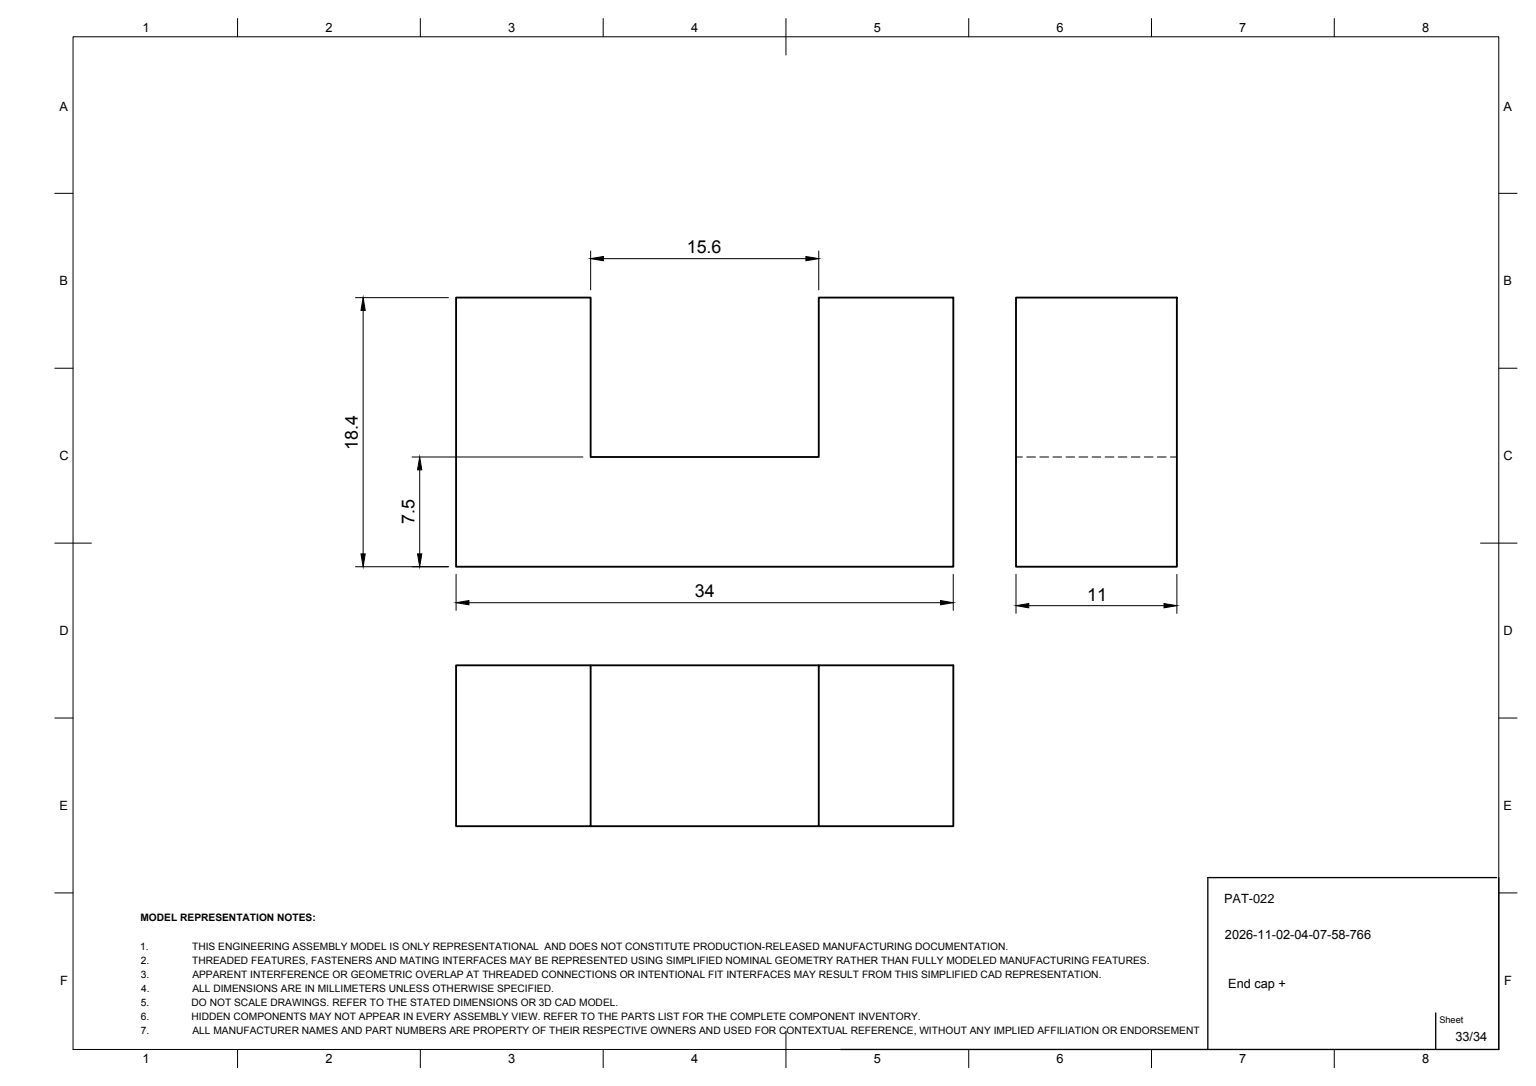
ISO-10303-21;
HEADER;
/* Generated by software containing ST-Developer
 * from STEP Tools, Inc. (www.steptools.com) 
 */

FILE_DESCRIPTION(
/* description */ ('Chute with adjustable gate'),
/* implementation_level */ '2;1');

FILE_NAME(
/* name */ 'End cap +.step',
/* time_stamp */ '2026-10-27T10:52:28-07:00',
/* author */ (''),
/* organization */ (''),
/* preprocessor_version */ 'ST-DEVELOPER v20.2',
/* originating_system */ 'Autodesk Translation Framework v15.17.0.0',
/* authorisation */ '');

FILE_SCHEMA (('AUTOMOTIVE_DESIGN { 1 0 10303 214 3 1 1 }'));
ENDSEC;

DATA;
#10=MECHANICAL_DESIGN_GEOMETRIC_PRESENTATION_REPRESENTATION('',(#442),#13094);
#378=SHAPE_REPRESENTATION_RELATIONSHIP('SRR','None',#13281,#410);
#410=ADVANCED_BREP_SHAPE_REPRESENTATION('',(#472),#13090);
#442=STYLED_ITEM('',(#13488),#472);
#472=MANIFOLD_SOLID_BREP('Body1',#7627);
#872=PLANE('',#8549);
#873=PLANE('',#8550);
#874=PLANE('',#8551);
#875=PLANE('',#8552);
#876=PLANE('',#8553);
#877=PLANE('',#8554);
#878=PLANE('',#8555);
#879=PLANE('',#8556);
#880=PLANE('',#8557);
#881=PLANE('',#8558);
#1276=FACE_OUTER_BOUND('',#1805,.T.);
#1277=FACE_OUTER_BOUND('',#1806,.T.);
#1278=FACE_OUTER_BOUND('',#1807,.T.);
#1279=FACE_OUTER_BOUND('',#1808,.T.);
#1280=FACE_OUTER_BOUND('',#1809,.T.);
#1281=FACE_OUTER_BOUND('',#1810,.T.);
#1282=FACE_OUTER_BOUND('',#1811,.T.);
#1283=FACE_OUTER_BOUND('',#1812,.T.);
#1284=FACE_OUTER_BOUND('',#1813,.T.);
#1285=FACE_OUTER_BOUND('',#1814,.T.);
#1805=EDGE_LOOP('',(#6886,#6887,#6888,#6889));
#1806=EDGE_LOOP('',(#6890,#6891,#6892,#6893));
#1807=EDGE_LOOP('',(#6894,#6895,#6896,#6897));
#1808=EDGE_LOOP('',(#6898,#6899,#6900,#6901));
#1809=EDGE_LOOP('',(#6902,#6903,#6904,#6905));
#1810=EDGE_LOOP('',(#6906,#6907,#6908,#6909));
#1811=EDGE_LOOP('',(#6910,#6911,#6912,#6913));
#1812=EDGE_LOOP('',(#6914,#6915,#6916,#6917));
#1813=EDGE_LOOP('',(#6918,#6919,#6920,#6921,#6922,#6923,#6924,#6925));
#1814=EDGE_LOOP('',(#6926,#6927,#6928,#6929,#6930,#6931,#6932,#6933));
#2542=LINE('',#12709,#3319);
#2543=LINE('',#12711,#3320);
#2544=LINE('',#12713,#3321);
#2545=LINE('',#12714,#3322);
#2546=LINE('',#12717,#3323);
#2547=LINE('',#12719,#3324);
#2548=LINE('',#12720,#3325);
#2549=LINE('',#12723,#3326);
#2550=LINE('',#12725,#3327);
#2551=LINE('',#12726,#3328);
#2552=LINE('',#12729,#3329);
#2553=LINE('',#12731,#3330);
#2554=LINE('',#12732,#3331);
#2555=LINE('',#12735,#3332);
#2556=LINE('',#12737,#3333);
#2557=LINE('',#12738,#3334);
#2558=LINE('',#12741,#3335);
#2559=LINE('',#12743,#3336);
#2560=LINE('',#12744,#3337);
#2561=LINE('',#12747,#3338);
#2562=LINE('',#12749,#3339);
#2563=LINE('',#12750,#3340);
#2564=LINE('',#12752,#3341);
#2565=LINE('',#12753,#3342);
#3319=VECTOR('',#10508,1.);
#3320=VECTOR('',#10509,1.);
#3321=VECTOR('',#10510,1.);
#3322=VECTOR('',#10511,1.);
#3323=VECTOR('',#10514,1.);
#3324=VECTOR('',#10515,1.);
#3325=VECTOR('',#10516,1.);
#3326=VECTOR('',#10519,1.);
#3327=VECTOR('',#10520,1.);
#3328=VECTOR('',#10521,1.);
#3329=VECTOR('',#10524,1.);
#3330=VECTOR('',#10525,1.);
#3331=VECTOR('',#10526,1.);
#3332=VECTOR('',#10529,1.);
#3333=VECTOR('',#10530,1.);
#3334=VECTOR('',#10531,1.);
#3335=VECTOR('',#10534,1.);
#3336=VECTOR('',#10535,1.);
#3337=VECTOR('',#10536,1.);
#3338=VECTOR('',#10539,1.);
#3339=VECTOR('',#10540,1.);
#3340=VECTOR('',#10541,1.);
#3341=VECTOR('',#10544,1.);
#3342=VECTOR('',#10545,1.);
#4155=VERTEX_POINT('',#12707);
#4156=VERTEX_POINT('',#12708);
#4157=VERTEX_POINT('',#12710);
#4158=VERTEX_POINT('',#12712);
#4159=VERTEX_POINT('',#12716);
#4160=VERTEX_POINT('',#12718);
#4161=VERTEX_POINT('',#12722);
#4162=VERTEX_POINT('',#12724);
#4163=VERTEX_POINT('',#12728);
#4164=VERTEX_POINT('',#12730);
#4165=VERTEX_POINT('',#12734);
#4166=VERTEX_POINT('',#12736);
#4167=VERTEX_POINT('',#12740);
#4168=VERTEX_POINT('',#12742);
#4169=VERTEX_POINT('',#12746);
#4170=VERTEX_POINT('',#12748);
#5076=EDGE_CURVE('',#4155,#4156,#2542,.T.);
#5077=EDGE_CURVE('',#4156,#4157,#2543,.T.);
#5078=EDGE_CURVE('',#4158,#4157,#2544,.T.);
#5079=EDGE_CURVE('',#4155,#4158,#2545,.T.);
#5080=EDGE_CURVE('',#4159,#4155,#2546,.T.);
#5081=EDGE_CURVE('',#4160,#4158,#2547,.T.);
#5082=EDGE_CURVE('',#4159,#4160,#2548,.T.);
#5083=EDGE_CURVE('',#4161,#4159,#2549,.T.);
#5084=EDGE_CURVE('',#4162,#4160,#2550,.T.);
#5085=EDGE_CURVE('',#4161,#4162,#2551,.T.);
#5086=EDGE_CURVE('',#4163,#4161,#2552,.T.);
#5087=EDGE_CURVE('',#4164,#4162,#2553,.T.);
#5088=EDGE_CURVE('',#4163,#4164,#2554,.T.);
#5089=EDGE_CURVE('',#4165,#4163,#2555,.T.);
#5090=EDGE_CURVE('',#4166,#4164,#2556,.T.);
#5091=EDGE_CURVE('',#4165,#4166,#2557,.T.);
#5092=EDGE_CURVE('',#4167,#4165,#2558,.T.);
#5093=EDGE_CURVE('',#4168,#4166,#2559,.T.);
#5094=EDGE_CURVE('',#4167,#4168,#2560,.T.);
#5095=EDGE_CURVE('',#4169,#4167,#2561,.T.);
#5096=EDGE_CURVE('',#4170,#4168,#2562,.T.);
#5097=EDGE_CURVE('',#4169,#4170,#2563,.T.);
#5098=EDGE_CURVE('',#4156,#4169,#2564,.T.);
#5099=EDGE_CURVE('',#4157,#4170,#2565,.T.);
#6886=ORIENTED_EDGE('',*,*,#5076,.T.);
#6887=ORIENTED_EDGE('',*,*,#5077,.T.);
#6888=ORIENTED_EDGE('',*,*,#5078,.F.);
#6889=ORIENTED_EDGE('',*,*,#5079,.F.);
#6890=ORIENTED_EDGE('',*,*,#5080,.T.);
#6891=ORIENTED_EDGE('',*,*,#5079,.T.);
#6892=ORIENTED_EDGE('',*,*,#5081,.F.);
#6893=ORIENTED_EDGE('',*,*,#5082,.F.);
#6894=ORIENTED_EDGE('',*,*,#5083,.T.);
#6895=ORIENTED_EDGE('',*,*,#5082,.T.);
#6896=ORIENTED_EDGE('',*,*,#5084,.F.);
#6897=ORIENTED_EDGE('',*,*,#5085,.F.);
#6898=ORIENTED_EDGE('',*,*,#5086,.T.);
#6899=ORIENTED_EDGE('',*,*,#5085,.T.);
#6900=ORIENTED_EDGE('',*,*,#5087,.F.);
#6901=ORIENTED_EDGE('',*,*,#5088,.F.);
#6902=ORIENTED_EDGE('',*,*,#5089,.T.);
#6903=ORIENTED_EDGE('',*,*,#5088,.T.);
#6904=ORIENTED_EDGE('',*,*,#5090,.F.);
#6905=ORIENTED_EDGE('',*,*,#5091,.F.);
#6906=ORIENTED_EDGE('',*,*,#5092,.T.);
#6907=ORIENTED_EDGE('',*,*,#5091,.T.);
#6908=ORIENTED_EDGE('',*,*,#5093,.F.);
#6909=ORIENTED_EDGE('',*,*,#5094,.F.);
#6910=ORIENTED_EDGE('',*,*,#5095,.T.);
#6911=ORIENTED_EDGE('',*,*,#5094,.T.);
#6912=ORIENTED_EDGE('',*,*,#5096,.F.);
#6913=ORIENTED_EDGE('',*,*,#5097,.F.);
#6914=ORIENTED_EDGE('',*,*,#5098,.T.);
#6915=ORIENTED_EDGE('',*,*,#5097,.T.);
#6916=ORIENTED_EDGE('',*,*,#5099,.F.);
#6917=ORIENTED_EDGE('',*,*,#5077,.F.);
#6918=ORIENTED_EDGE('',*,*,#5099,.T.);
#6919=ORIENTED_EDGE('',*,*,#5096,.T.);
#6920=ORIENTED_EDGE('',*,*,#5093,.T.);
#6921=ORIENTED_EDGE('',*,*,#5090,.T.);
#6922=ORIENTED_EDGE('',*,*,#5087,.T.);
#6923=ORIENTED_EDGE('',*,*,#5084,.T.);
#6924=ORIENTED_EDGE('',*,*,#5081,.T.);
#6925=ORIENTED_EDGE('',*,*,#5078,.T.);
#6926=ORIENTED_EDGE('',*,*,#5098,.F.);
#6927=ORIENTED_EDGE('',*,*,#5076,.F.);
#6928=ORIENTED_EDGE('',*,*,#5080,.F.);
#6929=ORIENTED_EDGE('',*,*,#5083,.F.);
#6930=ORIENTED_EDGE('',*,*,#5086,.F.);
#6931=ORIENTED_EDGE('',*,*,#5089,.F.);
#6932=ORIENTED_EDGE('',*,*,#5092,.F.);
#6933=ORIENTED_EDGE('',*,*,#5095,.F.);
#7544=ADVANCED_FACE('',(#1276),#872,.T.);
#7545=ADVANCED_FACE('',(#1277),#873,.T.);
#7546=ADVANCED_FACE('',(#1278),#874,.T.);
#7547=ADVANCED_FACE('',(#1279),#875,.T.);
#7548=ADVANCED_FACE('',(#1280),#876,.T.);
#7549=ADVANCED_FACE('',(#1281),#877,.T.);
#7550=ADVANCED_FACE('',(#1282),#878,.T.);
#7551=ADVANCED_FACE('',(#1283),#879,.T.);
#7552=ADVANCED_FACE('',(#1284),#880,.T.);
#7553=ADVANCED_FACE('',(#1285),#881,.F.);
#7627=CLOSED_SHELL('',(#7544,#7545,#7546,#7547,#7548,#7549,#7550,#7551,
#7552,#7553));
#8548=AXIS2_PLACEMENT_3D('',#12705,#10504,#10505);
#8549=AXIS2_PLACEMENT_3D('',#12706,#10506,#10507);
#8550=AXIS2_PLACEMENT_3D('',#12715,#10512,#10513);
#8551=AXIS2_PLACEMENT_3D('',#12721,#10517,#10518);
#8552=AXIS2_PLACEMENT_3D('',#12727,#10522,#10523);
#8553=AXIS2_PLACEMENT_3D('',#12733,#10527,#10528);
#8554=AXIS2_PLACEMENT_3D('',#12739,#10532,#10533);
#8555=AXIS2_PLACEMENT_3D('',#12745,#10537,#10538);
#8556=AXIS2_PLACEMENT_3D('',#12751,#10542,#10543);
#8557=AXIS2_PLACEMENT_3D('',#12754,#10546,#10547);
#8558=AXIS2_PLACEMENT_3D('',#12755,#10548,#10549);
#10504=DIRECTION('axis',(0.,0.,1.));
#10505=DIRECTION('refdir',(1.,0.,0.));
#10506=DIRECTION('center_axis',(0.,0.,1.));
#10507=DIRECTION('ref_axis',(0.,-1.,0.));
#10508=DIRECTION('',(0.,-1.,0.));
#10509=DIRECTION('',(1.,0.,0.));
#10510=DIRECTION('',(0.,-1.,0.));
#10511=DIRECTION('',(1.,0.,0.));
#10512=DIRECTION('center_axis',(0.,1.,0.));
#10513=DIRECTION('ref_axis',(0.,0.,1.));
#10514=DIRECTION('',(0.,0.,1.));
#10515=DIRECTION('',(0.,0.,1.));
#10516=DIRECTION('',(1.,0.,0.));
#10517=DIRECTION('center_axis',(0.,0.,-1.));
#10518=DIRECTION('ref_axis',(0.,1.,0.));
#10519=DIRECTION('',(0.,1.,0.));
#10520=DIRECTION('',(0.,1.,0.));
#10521=DIRECTION('',(1.,0.,0.));
#10522=DIRECTION('center_axis',(0.,-1.,0.));
#10523=DIRECTION('ref_axis',(0.,0.,-1.));
#10524=DIRECTION('',(0.,0.,-1.));
#10525=DIRECTION('',(0.,0.,-1.));
#10526=DIRECTION('',(1.,0.,0.));
#10527=DIRECTION('center_axis',(0.,0.,-1.));
#10528=DIRECTION('ref_axis',(0.,1.,0.));
#10529=DIRECTION('',(0.,1.,0.));
#10530=DIRECTION('',(0.,1.,0.));
#10531=DIRECTION('',(1.,0.,0.));
#10532=DIRECTION('center_axis',(0.,1.,0.));
#10533=DIRECTION('ref_axis',(0.,0.,1.));
#10534=DIRECTION('',(0.,0.,1.));
#10535=DIRECTION('',(0.,0.,1.));
#10536=DIRECTION('',(1.,0.,0.));
#10537=DIRECTION('center_axis',(0.,0.,-1.));
#10538=DIRECTION('ref_axis',(0.,1.,0.));
#10539=DIRECTION('',(0.,1.,0.));
#10540=DIRECTION('',(0.,1.,0.));
#10541=DIRECTION('',(1.,0.,0.));
#10542=DIRECTION('center_axis',(0.,-1.,0.));
#10543=DIRECTION('ref_axis',(0.,0.,-1.));
#10544=DIRECTION('',(0.,0.,-1.));
#10545=DIRECTION('',(0.,0.,-1.));
#10546=DIRECTION('center_axis',(1.,0.,0.));
#10547=DIRECTION('ref_axis',(0.,0.,-1.));
#10548=DIRECTION('center_axis',(1.,0.,0.));
#10549=DIRECTION('ref_axis',(0.,0.,-1.));
#12705=CARTESIAN_POINT('',(0.,0.,0.));
#12706=CARTESIAN_POINT('Origin',(1.97,1.7,2.3));
#12707=CARTESIAN_POINT('',(1.97,1.7,2.3));
#12708=CARTESIAN_POINT('',(1.97,-1.7,2.3));
#12709=CARTESIAN_POINT('',(1.97,1.7,2.3));
#12710=CARTESIAN_POINT('',(3.07,-1.7,2.3));
#12711=CARTESIAN_POINT('',(1.97,-1.7,2.3));
#12712=CARTESIAN_POINT('',(3.07,1.7,2.3));
#12713=CARTESIAN_POINT('',(3.07,1.7,2.3));
#12714=CARTESIAN_POINT('',(1.97,1.7,2.3));
#12715=CARTESIAN_POINT('Origin',(1.97,1.7,0.46));
#12716=CARTESIAN_POINT('',(1.97,1.7,0.46));
#12717=CARTESIAN_POINT('',(1.97,1.7,0.46));
#12718=CARTESIAN_POINT('',(3.07,1.7,0.46));
#12719=CARTESIAN_POINT('',(3.07,1.7,0.46));
#12720=CARTESIAN_POINT('',(1.97,1.7,0.46));
#12721=CARTESIAN_POINT('Origin',(1.97,0.78,0.46));
#12722=CARTESIAN_POINT('',(1.97,0.78,0.46));
#12723=CARTESIAN_POINT('',(1.97,0.78,0.46));
#12724=CARTESIAN_POINT('',(3.07,0.78,0.46));
#12725=CARTESIAN_POINT('',(3.07,0.78,0.46));
#12726=CARTESIAN_POINT('',(1.97,0.78,0.46));
#12727=CARTESIAN_POINT('Origin',(1.97,0.78,1.55));
#12728=CARTESIAN_POINT('',(1.97,0.78,1.55));
#12729=CARTESIAN_POINT('',(1.97,0.78,1.55));
#12730=CARTESIAN_POINT('',(3.07,0.78,1.55));
#12731=CARTESIAN_POINT('',(3.07,0.78,1.55));
#12732=CARTESIAN_POINT('',(1.97,0.78,1.55));
#12733=CARTESIAN_POINT('Origin',(1.97,-0.78,1.55));
#12734=CARTESIAN_POINT('',(1.97,-0.78,1.55));
#12735=CARTESIAN_POINT('',(1.97,-0.78,1.55));
#12736=CARTESIAN_POINT('',(3.07,-0.78,1.55));
#12737=CARTESIAN_POINT('',(3.07,-0.78,1.55));
#12738=CARTESIAN_POINT('',(1.97,-0.78,1.55));
#12739=CARTESIAN_POINT('Origin',(1.97,-0.78,0.46));
#12740=CARTESIAN_POINT('',(1.97,-0.78,0.46));
#12741=CARTESIAN_POINT('',(1.97,-0.78,0.46));
#12742=CARTESIAN_POINT('',(3.07,-0.78,0.46));
#12743=CARTESIAN_POINT('',(3.07,-0.78,0.46));
#12744=CARTESIAN_POINT('',(1.97,-0.78,0.46));
#12745=CARTESIAN_POINT('Origin',(1.97,-1.7,0.46));
#12746=CARTESIAN_POINT('',(1.97,-1.7,0.46));
#12747=CARTESIAN_POINT('',(1.97,-1.7,0.46));
#12748=CARTESIAN_POINT('',(3.07,-1.7,0.46));
#12749=CARTESIAN_POINT('',(3.07,-1.7,0.46));
#12750=CARTESIAN_POINT('',(1.97,-1.7,0.46));
#12751=CARTESIAN_POINT('Origin',(1.97,-1.7,2.3));
#12752=CARTESIAN_POINT('',(1.97,-1.7,2.3));
#12753=CARTESIAN_POINT('',(3.07,-1.7,2.3));
#12754=CARTESIAN_POINT('Origin',(3.07,0.,1.38));
#12755=CARTESIAN_POINT('Origin',(1.97,0.,1.38));
#13053=UNCERTAINTY_MEASURE_WITH_UNIT(LENGTH_MEASURE(0.001),#13095,
'DISTANCE_ACCURACY_VALUE',
'Maximum model space distance between geometric entities at asserted c
onnectivities');
#13057=UNCERTAINTY_MEASURE_WITH_UNIT(LENGTH_MEASURE(0.001),#13095,
'DISTANCE_ACCURACY_VALUE',
'Maximum model space distance between geometric entities at asserted c
onnectivities');
#13090=(
GEOMETRIC_REPRESENTATION_CONTEXT(3)
GLOBAL_UNCERTAINTY_ASSIGNED_CONTEXT((#13053))
GLOBAL_UNIT_ASSIGNED_CONTEXT((#13095,#13097,#13098))
REPRESENTATION_CONTEXT('','3D')
);
#13094=(
GEOMETRIC_REPRESENTATION_CONTEXT(3)
GLOBAL_UNCERTAINTY_ASSIGNED_CONTEXT((#13057))
GLOBAL_UNIT_ASSIGNED_CONTEXT((#13095,#13097,#13098))
REPRESENTATION_CONTEXT('','3D')
);
#13095=(
LENGTH_UNIT()
NAMED_UNIT(*)
SI_UNIT(.CENTI.,.METRE.)
);
#13097=(
NAMED_UNIT(*)
PLANE_ANGLE_UNIT()
SI_UNIT($,.RADIAN.)
);
#13098=(
NAMED_UNIT(*)
SI_UNIT($,.STERADIAN.)
SOLID_ANGLE_UNIT()
);
#13131=SHAPE_DEFINITION_REPRESENTATION(#13167,#13281);
#13167=PRODUCT_DEFINITION_SHAPE('',$,#13318);
#13281=SHAPE_REPRESENTATION('',(#8548),#13090);
#13285=PRODUCT_DEFINITION_CONTEXT('part definition',#13395,'design');
#13318=PRODUCT_DEFINITION('End cap +','End cap +',#13354,#13285);
#13354=PRODUCT_DEFINITION_FORMATION('',$,#13429);
#13395=APPLICATION_CONTEXT(
'Core Data for Automotive Mechanical Design Process');
#13396=PRODUCT_CONTEXT('part definition',#13395,'mechanical');
#13429=PRODUCT('End cap +','End cap +','End cap +',(#13396));
#13482=COLOUR_RGB('Sky Blue',0.24,0.69,0.87);
#13483=FILL_AREA_STYLE_COLOUR('',#13482);
#13484=FILL_AREA_STYLE('',(#13483));
#13485=SURFACE_STYLE_FILL_AREA(#13484);
#13486=SURFACE_SIDE_STYLE('',(#13485));
#13487=SURFACE_STYLE_USAGE(.BOTH.,#13486);
#13488=PRESENTATION_STYLE_ASSIGNMENT((#13487));
ENDSEC;
END-ISO-10303-21;
